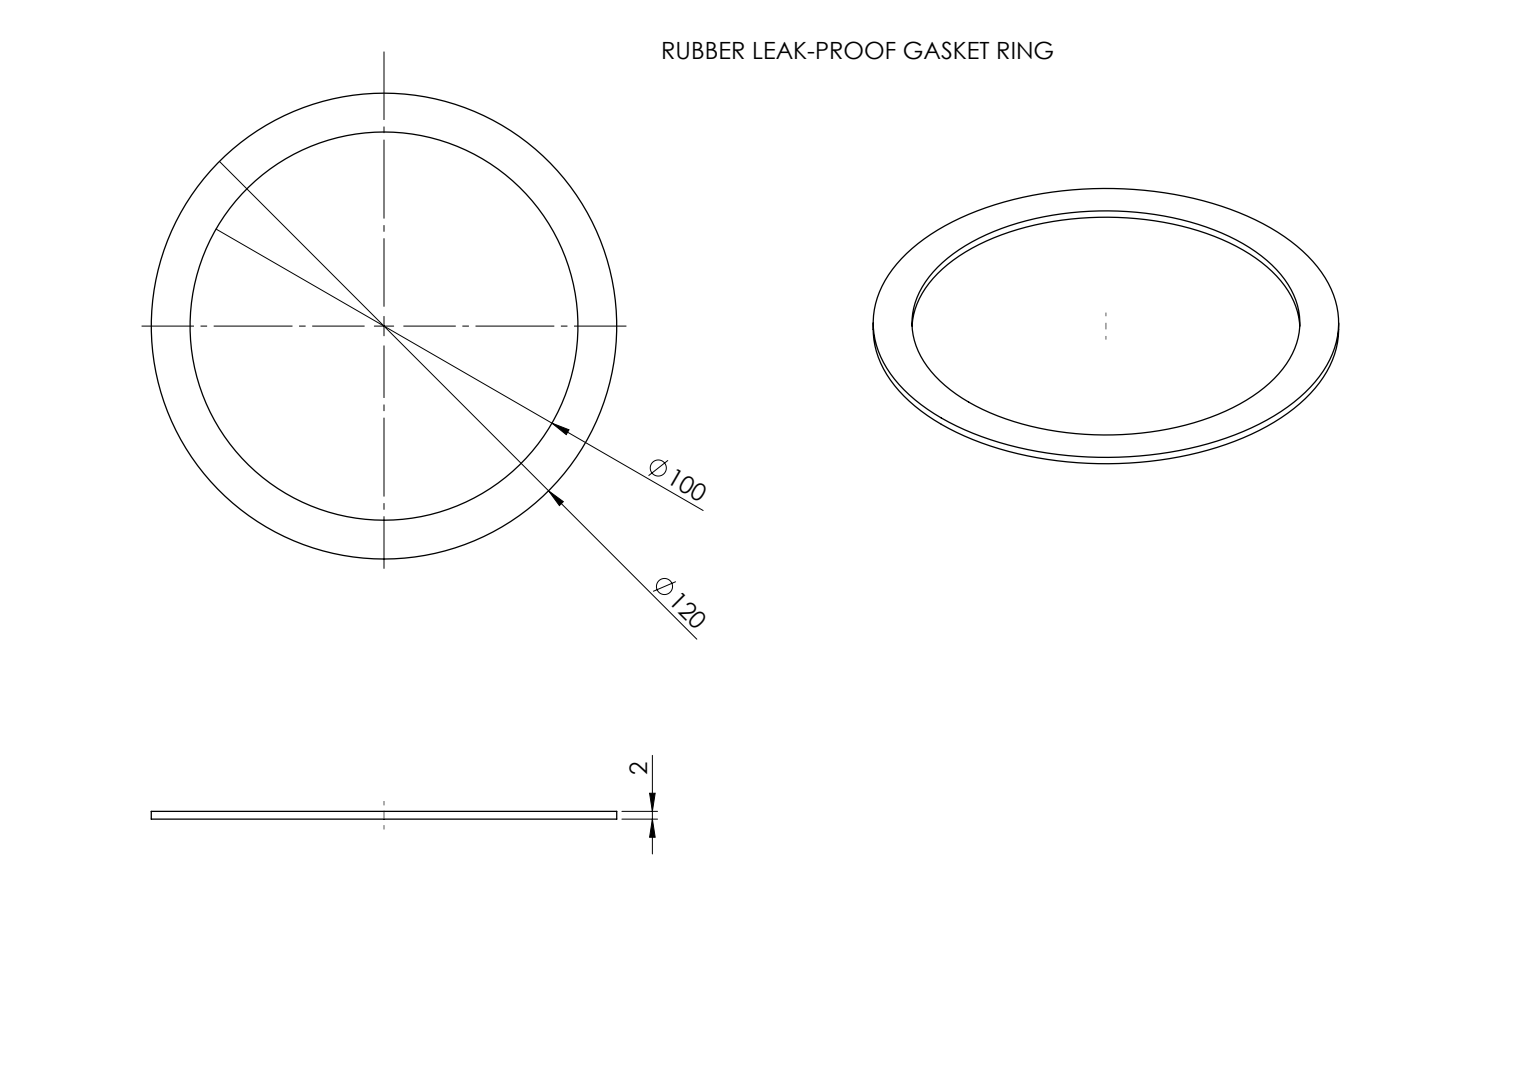
ISO-10303-21;
HEADER;
FILE_DESCRIPTION (('STEP AP214'),
    '1' );
FILE_NAME ('Rubber Leak-Proof Gasket Ring.step',
    '2026-10-09T15:02:13',
    ( '' ),
    ( '' ),
    'SwSTEP 2.0',
    'SolidWorks 2026',
    '' );
FILE_SCHEMA (( 'AUTOMOTIVE_DESIGN' ));
ENDSEC;

DATA;
#75=VERTEX_POINT ( 'NONE', #14029 ) ;
#118=ORIENTED_EDGE ( 'NONE', *, *, #603, .F. ) ;
#141=DIRECTION ( 'NONE',  ( 0.000000000000000000, 0.000000000000000000, -1.000000000000000000 ) ) ;
#205=EDGE_CURVE ( 'NONE', #75, #14665, #7073, .T. ) ;
#230=DIRECTION ( 'NONE',  ( 0.000000000000000000, 0.000000000000000000, 1.000000000000000000 ) ) ;
#240=DIRECTION ( 'NONE',  ( 0.000000000000000000, 1.000000000000000000, 0.000000000000000000 ) ) ;
#243=VERTEX_POINT ( 'NONE', #6253 ) ;
#295=PRODUCT_DEFINITION ( 'UNKNOWN', '', #14486, #8928 ) ;
#378=FACE_OUTER_BOUND ( 'NONE', #6121, .T. ) ;
#382=CARTESIAN_POINT ( 'NONE',  ( 0.000000000000000000, 52.00000000000000711, 0.000000000000000000 ) ) ;
#550=DIRECTION ( 'NONE',  ( 0.000000000000000000, 1.000000000000000000, 0.000000000000000000 ) ) ;
#603=EDGE_CURVE ( 'NONE', #14587, #8799, #10009, .T. ) ;
#730=SHAPE_REPRESENTATION_RELATIONSHIP ( 'NONE' , 'NONE' ,  #15829, #9194 ) ;
#848=DIRECTION ( 'NONE',  ( 0.000000000000000000, 0.000000000000000000, 1.000000000000000000 ) ) ;
#911=CYLINDRICAL_SURFACE ( 'NONE', #979, 50.00000000000000000 ) ;
#976=( LENGTH_UNIT ( ) NAMED_UNIT ( * ) SI_UNIT ( .MILLI., .METRE. ) );
#979=AXIS2_PLACEMENT_3D ( 'NONE', #3337, #9656, #12404 ) ;
#1079=ADVANCED_FACE ( 'NONE', ( #8408 ), #911, .F. ) ;
#1119=CIRCLE ( 'NONE', #15991, 50.00000000000000000 ) ;
#1131=AXIS2_PLACEMENT_3D ( 'NONE', #1874, #6969, #10701 ) ;
#1133=( NAMED_UNIT ( * ) PLANE_ANGLE_UNIT ( ) SI_UNIT ( $, .RADIAN. ) );
#1217=CIRCLE ( 'NONE', #4436, 50.00000000000000000 ) ;
#1229=EDGE_CURVE ( 'NONE', #8799, #14587, #16125, .T. ) ;
#1243=CIRCLE ( 'NONE', #5001, 50.00000000000000000 ) ;
#1279=CARTESIAN_POINT ( 'NONE',  ( 0.000000000000000000, 50.00000000000000000, 0.000000000000000000 ) ) ;
#1353=ORIENTED_EDGE ( 'NONE', *, *, #4912, .T. ) ;
#1385=CARTESIAN_POINT ( 'NONE',  ( 0.000000000000000000, 52.00000000000000711, -60.00000000000000711 ) ) ;
#1481=DIRECTION ( 'NONE',  ( -0.000000000000000000, -1.000000000000000000, -0.000000000000000000 ) ) ;
#1534=ADVANCED_FACE ( 'NONE', ( #5816, #3149 ), #10883, .T. ) ;
#1684=EDGE_CURVE ( 'NONE', #8698, #14922, #1243, .T. ) ;
#1738=( GEOMETRIC_REPRESENTATION_CONTEXT ( 3 ) GLOBAL_UNCERTAINTY_ASSIGNED_CONTEXT ( ( #14556 ) ) GLOBAL_UNIT_ASSIGNED_CONTEXT ( ( #9391, #6750, #13366 ) ) REPRESENTATION_CONTEXT ( 'NONE', 'WORKASPACE' ) );
#1874=CARTESIAN_POINT ( 'NONE',  ( 0.000000000000000000, 52.00000000000000711, 0.000000000000000000 ) ) ;
#1973=ORIENTED_EDGE ( 'NONE', *, *, #10109, .F. ) ;
#2000=EDGE_LOOP ( 'NONE', ( #3155, #11326, #2184, #1973 ) ) ;
#2077=APPLICATION_CONTEXT ( 'automotive_design' ) ;
#2158=CARTESIAN_POINT ( 'NONE',  ( 0.000000000000000000, 0.000000000000000000, 0.000000000000000000 ) ) ;
#2184=ORIENTED_EDGE ( 'NONE', *, *, #1684, .F. ) ;
#2306=AXIS2_PLACEMENT_3D ( 'NONE', #10308, #1481, #141 ) ;
#2469=VECTOR ( 'NONE', #6768, 1000.000000000000000 ) ;
#2506=LINE ( 'NONE', #11570, #11062 ) ;
#2528=PLANE ( 'NONE',  #6500 ) ;
#2581=AXIS2_PLACEMENT_3D ( 'NONE', #15699, #240, #10476 ) ;
#2725=CYLINDRICAL_SURFACE ( 'NONE', #2306, 60.00000000000000711 ) ;
#2829=DIRECTION ( 'NONE',  ( 0.000000000000000000, 1.000000000000000000, 0.000000000000000000 ) ) ;
#2954=ORIENTED_EDGE ( 'NONE', *, *, #14421, .T. ) ;
#3147=( NAMED_UNIT ( * ) PLANE_ANGLE_UNIT ( ) SI_UNIT ( $, .RADIAN. ) );
#3149=FACE_BOUND ( 'NONE', #5769, .T. ) ;
#3155=ORIENTED_EDGE ( 'NONE', *, *, #4858, .T. ) ;
#3337=CARTESIAN_POINT ( 'NONE',  ( 0.000000000000000000, 52.00000000000000711, 0.000000000000000000 ) ) ;
#3399=ADVANCED_FACE ( 'NONE', ( #10311 ), #8889, .F. ) ;
#3554=ORIENTED_EDGE ( 'NONE', *, *, #14421, .F. ) ;
#3656=SURFACE_STYLE_FILL_AREA ( #12620 ) ;
#3680=DIRECTION ( 'NONE',  ( 0.000000000000000000, 1.000000000000000000, 0.000000000000000000 ) ) ;
#3792=MECHANICAL_DESIGN_GEOMETRIC_PRESENTATION_REPRESENTATION('',(#10950),#14656);
#3875=STYLED_ITEM ( 'NONE', ( #9556 ), #9194 ) ;
#3944=ORIENTED_EDGE ( 'NONE', *, *, #12365, .F. ) ;
#4056=COLOUR_RGB ( '', 0.66274510, 0.83137255, 0.94901961) ;
#4226=SHAPE_DEFINITION_REPRESENTATION ( #11839, #15829 ) ;
#4230=DIRECTION ( 'NONE',  ( 0.000000000000000000, 0.000000000000000000, -1.000000000000000000 ) ) ;
#4436=AXIS2_PLACEMENT_3D ( 'NONE', #9671, #7184, #848 ) ;
#4466=LINE ( 'NONE', #9443, #4960 ) ;
#4525=ORIENTED_EDGE ( 'NONE', *, *, #205, .F. ) ;
#4541=ORIENTED_EDGE ( 'NONE', *, *, #14844, .T. ) ;
#4715=AXIS2_PLACEMENT_3D ( 'NONE', #13895, #6517, #10172 ) ;
#4752=( NAMED_UNIT ( * ) SI_UNIT ( $, .STERADIAN. ) SOLID_ANGLE_UNIT ( ) );
#4828=FILL_AREA_STYLE ('',( #13533 ) ) ;
#4858=EDGE_CURVE ( 'NONE', #243, #15421, #1217, .T. ) ;
#4912=EDGE_CURVE ( 'NONE', #14665, #14587, #2506, .T. ) ;
#4960=VECTOR ( 'NONE', #6023, 1000.000000000000000 ) ;
#5001=AXIS2_PLACEMENT_3D ( 'NONE', #5654, #2829, #13215 ) ;
#5190=CARTESIAN_POINT ( 'NONE',  ( 6.123233995736766085E-15, 52.00000000000000711, 50.00000000000000000 ) ) ;
#5227=CLOSED_SHELL ( 'NONE', ( #3399, #12072, #1534, #7840, #14756, #1079 ) ) ;
#5446=ORIENTED_EDGE ( 'NONE', *, *, #12365, .T. ) ;
#5480=CYLINDRICAL_SURFACE ( 'NONE', #14924, 60.00000000000000711 ) ;
#5621=PRODUCT ( 'Rubber Leak-Proof Gasket Ring', 'Rubber Leak-Proof Gasket Ring', '', ( #10375 ) ) ;
#5654=CARTESIAN_POINT ( 'NONE',  ( 0.000000000000000000, 50.00000000000000000, 0.000000000000000000 ) ) ;
#5769=EDGE_LOOP ( 'NONE', ( #6079, #3944 ) ) ;
#5816=FACE_OUTER_BOUND ( 'NONE', #9542, .T. ) ;
#5897=( NAMED_UNIT ( * ) SI_UNIT ( $, .STERADIAN. ) SOLID_ANGLE_UNIT ( ) );
#5982=DIRECTION ( 'NONE',  ( 0.000000000000000000, 1.000000000000000000, 0.000000000000000000 ) ) ;
#6023=DIRECTION ( 'NONE',  ( -0.000000000000000000, -1.000000000000000000, -0.000000000000000000 ) ) ;
#6071=SURFACE_SIDE_STYLE ('',( #14856 ) ) ;
#6079=ORIENTED_EDGE ( 'NONE', *, *, #4858, .F. ) ;
#6121=EDGE_LOOP ( 'NONE', ( #7382, #6800, #1353, #10798 ) ) ;
#6149=SURFACE_STYLE_USAGE ( .BOTH. , #12538 ) ;
#6253=CARTESIAN_POINT ( 'NONE',  ( 0.000000000000000000, 52.00000000000000711, -50.00000000000000000 ) ) ;
#6369=DIRECTION ( 'NONE',  ( 0.000000000000000000, 1.000000000000000000, 0.000000000000000000 ) ) ;
#6500=AXIS2_PLACEMENT_3D ( 'NONE', #1279, #6369, #10186 ) ;
#6517=DIRECTION ( 'NONE',  ( 0.000000000000000000, 1.000000000000000000, 0.000000000000000000 ) ) ;
#6573=EDGE_LOOP ( 'NONE', ( #118, #13201 ) ) ;
#6615=UNCERTAINTY_MEASURE_WITH_UNIT (LENGTH_MEASURE( 1.000000000000000082E-05 ), #12209, 'distance_accuracy_value', 'NONE');
#6750=( NAMED_UNIT ( * ) PLANE_ANGLE_UNIT ( ) SI_UNIT ( $, .RADIAN. ) );
#6768=DIRECTION ( 'NONE',  ( -0.000000000000000000, -1.000000000000000000, -0.000000000000000000 ) ) ;
#6800=ORIENTED_EDGE ( 'NONE', *, *, #14844, .F. ) ;
#6969=DIRECTION ( 'NONE',  ( 0.000000000000000000, 1.000000000000000000, 0.000000000000000000 ) ) ;
#6984=CARTESIAN_POINT ( 'NONE',  ( 0.000000000000000000, 50.00000000000000000, 0.000000000000000000 ) ) ;
#7073=CIRCLE ( 'NONE', #11325, 60.00000000000000711 ) ;
#7100=UNCERTAINTY_MEASURE_WITH_UNIT (LENGTH_MEASURE( 1.000000000000000082E-05 ), #976, 'distance_accuracy_value', 'NONE');
#7184=DIRECTION ( 'NONE',  ( 0.000000000000000000, 1.000000000000000000, 0.000000000000000000 ) ) ;
#7228=FILL_AREA_STYLE_COLOUR ( '', #4056 ) ;
#7382=ORIENTED_EDGE ( 'NONE', *, *, #15572, .F. ) ;
#7475=ORIENTED_EDGE ( 'NONE', *, *, #1229, .T. ) ;
#7631=AXIS2_PLACEMENT_3D ( 'NONE', #7886, #550, #230 ) ;
#7828=LINE ( 'NONE', #12903, #2469 ) ;
#7840=ADVANCED_FACE ( 'NONE', ( #8849, #13909 ), #2528, .F. ) ;
#7865=EDGE_LOOP ( 'NONE', ( #4525, #11866, #7475, #14355 ) ) ;
#7886=CARTESIAN_POINT ( 'NONE',  ( 0.000000000000000000, 52.00000000000000711, 0.000000000000000000 ) ) ;
#7957=AXIS2_PLACEMENT_3D ( 'NONE', #12549, #12717, #15367 ) ;
#8006=DIRECTION ( 'NONE',  ( -0.000000000000000000, -1.000000000000000000, -0.000000000000000000 ) ) ;
#8178=LINE ( 'NONE', #10600, #15299 ) ;
#8221=SURFACE_STYLE_USAGE ( .BOTH. , #6071 ) ;
#8223=CARTESIAN_POINT ( 'NONE',  ( 0.000000000000000000, 52.00000000000000711, 0.000000000000000000 ) ) ;
#8312=CIRCLE ( 'NONE', #1131, 60.00000000000000711 ) ;
#8408=FACE_OUTER_BOUND ( 'NONE', #10218, .T. ) ;
#8560=DIRECTION ( 'NONE',  ( 1.000000000000000000, 0.000000000000000000, 0.000000000000000000 ) ) ;
#8698=VERTEX_POINT ( 'NONE', #10157 ) ;
#8799=VERTEX_POINT ( 'NONE', #9247 ) ;
#8849=FACE_OUTER_BOUND ( 'NONE', #6573, .T. ) ;
#8889=CYLINDRICAL_SURFACE ( 'NONE', #7957, 50.00000000000000000 ) ;
#8928=PRODUCT_DEFINITION_CONTEXT ( 'detailed design', #2077, 'design' ) ;
#9178=( GEOMETRIC_REPRESENTATION_CONTEXT ( 3 ) GLOBAL_UNCERTAINTY_ASSIGNED_CONTEXT ( ( #6615 ) ) GLOBAL_UNIT_ASSIGNED_CONTEXT ( ( #12209, #3147, #5897 ) ) REPRESENTATION_CONTEXT ( 'NONE', 'WORKASPACE' ) );
#9194=ADVANCED_BREP_SHAPE_REPRESENTATION ( '', ( #14597, #15812 ), #1738 ) ;
#9247=CARTESIAN_POINT ( 'NONE',  ( 7.347880794884119933E-15, 50.00000000000000000, 60.00000000000000711 ) ) ;
#9391=( LENGTH_UNIT ( ) NAMED_UNIT ( * ) SI_UNIT ( .MILLI., .METRE. ) );
#9443=CARTESIAN_POINT ( 'NONE',  ( 0.000000000000000000, 52.00000000000000711, -50.00000000000000000 ) ) ;
#9487=EDGE_LOOP ( 'NONE', ( #10083, #2954 ) ) ;
#9542=EDGE_LOOP ( 'NONE', ( #4541, #12694 ) ) ;
#9556=PRESENTATION_STYLE_ASSIGNMENT (( #8221 ) ) ;
#9656=DIRECTION ( 'NONE',  ( -0.000000000000000000, -1.000000000000000000, -0.000000000000000000 ) ) ;
#9671=CARTESIAN_POINT ( 'NONE',  ( 0.000000000000000000, 52.00000000000000711, 0.000000000000000000 ) ) ;
#9700=CARTESIAN_POINT ( 'NONE',  ( 6.123233995736766085E-15, 50.00000000000000000, 50.00000000000000000 ) ) ;
#9720=CIRCLE ( 'NONE', #7631, 50.00000000000000000 ) ;
#10009=CIRCLE ( 'NONE', #4715, 60.00000000000000711 ) ;
#10083=ORIENTED_EDGE ( 'NONE', *, *, #1684, .T. ) ;
#10109=EDGE_CURVE ( 'NONE', #243, #8698, #4466, .T. ) ;
#10157=CARTESIAN_POINT ( 'NONE',  ( 0.000000000000000000, 50.00000000000000000, -50.00000000000000000 ) ) ;
#10172=DIRECTION ( 'NONE',  ( 0.000000000000000000, 0.000000000000000000, 1.000000000000000000 ) ) ;
#10186=DIRECTION ( 'NONE',  ( 0.000000000000000000, -0.000000000000000000, 1.000000000000000000 ) ) ;
#10218=EDGE_LOOP ( 'NONE', ( #15788, #5446, #15922, #3554 ) ) ;
#10308=CARTESIAN_POINT ( 'NONE',  ( 0.000000000000000000, 52.00000000000000711, 0.000000000000000000 ) ) ;
#10311=FACE_OUTER_BOUND ( 'NONE', #2000, .T. ) ;
#10375=PRODUCT_CONTEXT ( 'NONE', #12159, 'mechanical' ) ;
#10476=DIRECTION ( 'NONE',  ( 0.000000000000000000, 0.000000000000000000, 1.000000000000000000 ) ) ;
#10552=CARTESIAN_POINT ( 'NONE',  ( 0.000000000000000000, 52.00000000000000711, 0.000000000000000000 ) ) ;
#10600=CARTESIAN_POINT ( 'NONE',  ( 6.123233995736766085E-15, 52.00000000000000711, 50.00000000000000000 ) ) ;
#10701=DIRECTION ( 'NONE',  ( 0.000000000000000000, 0.000000000000000000, 1.000000000000000000 ) ) ;
#10798=ORIENTED_EDGE ( 'NONE', *, *, #603, .T. ) ;
#10811=DIRECTION ( 'NONE',  ( 0.000000000000000000, 1.000000000000000000, 0.000000000000000000 ) ) ;
#10883=PLANE ( 'NONE',  #12938 ) ;
#10950=STYLED_ITEM ( 'NONE', ( #16122 ), #14597 ) ;
#11037=COLOUR_RGB ( '', 0.66274510, 0.83137255, 0.94901961) ;
#11062=VECTOR ( 'NONE', #15308, 1000.000000000000000 ) ;
#11073=DIRECTION ( 'NONE',  ( 0.000000000000000000, 0.000000000000000000, 1.000000000000000000 ) ) ;
#11104=EDGE_CURVE ( 'NONE', #15421, #14922, #8178, .T. ) ;
#11325=AXIS2_PLACEMENT_3D ( 'NONE', #382, #3680, #13721 ) ;
#11326=ORIENTED_EDGE ( 'NONE', *, *, #11104, .T. ) ;
#11390=FACE_OUTER_BOUND ( 'NONE', #7865, .T. ) ;
#11570=CARTESIAN_POINT ( 'NONE',  ( 0.000000000000000000, 52.00000000000000711, -60.00000000000000711 ) ) ;
#11839=PRODUCT_DEFINITION_SHAPE ( 'NONE', 'NONE',  #295 ) ;
#11866=ORIENTED_EDGE ( 'NONE', *, *, #15572, .T. ) ;
#12072=ADVANCED_FACE ( 'NONE', ( #11390 ), #2725, .T. ) ;
#12159=APPLICATION_CONTEXT ( 'automotive_design' ) ;
#12209=( LENGTH_UNIT ( ) NAMED_UNIT ( * ) SI_UNIT ( .MILLI., .METRE. ) );
#12365=EDGE_CURVE ( 'NONE', #15421, #243, #9720, .T. ) ;
#12404=DIRECTION ( 'NONE',  ( 0.000000000000000000, 0.000000000000000000, -1.000000000000000000 ) ) ;
#12464=CARTESIAN_POINT ( 'NONE',  ( 0.000000000000000000, 50.00000000000000000, -60.00000000000000711 ) ) ;
#12538=SURFACE_SIDE_STYLE ('',( #3656 ) ) ;
#12549=CARTESIAN_POINT ( 'NONE',  ( 0.000000000000000000, 52.00000000000000711, 0.000000000000000000 ) ) ;
#12620=FILL_AREA_STYLE ('',( #7228 ) ) ;
#12694=ORIENTED_EDGE ( 'NONE', *, *, #205, .T. ) ;
#12717=DIRECTION ( 'NONE',  ( -0.000000000000000000, -1.000000000000000000, -0.000000000000000000 ) ) ;
#12903=CARTESIAN_POINT ( 'NONE',  ( 7.347880794884119933E-15, 52.00000000000000711, 60.00000000000000711 ) ) ;
#12938=AXIS2_PLACEMENT_3D ( 'NONE', #8223, #5982, #13289 ) ;
#13159=MECHANICAL_DESIGN_GEOMETRIC_PRESENTATION_REPRESENTATION('',(#3875),#9178);
#13201=ORIENTED_EDGE ( 'NONE', *, *, #1229, .F. ) ;
#13215=DIRECTION ( 'NONE',  ( 0.000000000000000000, 0.000000000000000000, 1.000000000000000000 ) ) ;
#13289=DIRECTION ( 'NONE',  ( 0.000000000000000000, -0.000000000000000000, 1.000000000000000000 ) ) ;
#13366=( NAMED_UNIT ( * ) SI_UNIT ( $, .STERADIAN. ) SOLID_ANGLE_UNIT ( ) );
#13533=FILL_AREA_STYLE_COLOUR ( '', #11037 ) ;
#13721=DIRECTION ( 'NONE',  ( 0.000000000000000000, 0.000000000000000000, 1.000000000000000000 ) ) ;
#13895=CARTESIAN_POINT ( 'NONE',  ( 0.000000000000000000, 50.00000000000000000, 0.000000000000000000 ) ) ;
#13909=FACE_BOUND ( 'NONE', #9487, .T. ) ;
#14029=CARTESIAN_POINT ( 'NONE',  ( 7.347880794884119933E-15, 52.00000000000000711, 60.00000000000000711 ) ) ;
#14355=ORIENTED_EDGE ( 'NONE', *, *, #4912, .F. ) ;
#14421=EDGE_CURVE ( 'NONE', #14922, #8698, #1119, .T. ) ;
#14486=PRODUCT_DEFINITION_FORMATION_WITH_SPECIFIED_SOURCE ( 'ANY', '', #5621, .NOT_KNOWN. ) ;
#14556=UNCERTAINTY_MEASURE_WITH_UNIT (LENGTH_MEASURE( 1.000000000000000082E-05 ), #9391, 'distance_accuracy_value', 'NONE');
#14587=VERTEX_POINT ( 'NONE', #12464 ) ;
#14597=MANIFOLD_SOLID_BREP ( 'Boss-Extrude1', #5227 ) ;
#14656=( GEOMETRIC_REPRESENTATION_CONTEXT ( 3 ) GLOBAL_UNCERTAINTY_ASSIGNED_CONTEXT ( ( #7100 ) ) GLOBAL_UNIT_ASSIGNED_CONTEXT ( ( #976, #1133, #4752 ) ) REPRESENTATION_CONTEXT ( 'NONE', 'WORKASPACE' ) );
#14665=VERTEX_POINT ( 'NONE', #1385 ) ;
#14756=ADVANCED_FACE ( 'NONE', ( #378 ), #5480, .T. ) ;
#14844=EDGE_CURVE ( 'NONE', #14665, #75, #8312, .T. ) ;
#14856=SURFACE_STYLE_FILL_AREA ( #4828 ) ;
#14922=VERTEX_POINT ( 'NONE', #9700 ) ;
#14924=AXIS2_PLACEMENT_3D ( 'NONE', #10552, #15608, #4230 ) ;
#15299=VECTOR ( 'NONE', #8006, 1000.000000000000000 ) ;
#15308=DIRECTION ( 'NONE',  ( -0.000000000000000000, -1.000000000000000000, -0.000000000000000000 ) ) ;
#15367=DIRECTION ( 'NONE',  ( 0.000000000000000000, 0.000000000000000000, -1.000000000000000000 ) ) ;
#15421=VERTEX_POINT ( 'NONE', #5190 ) ;
#15572=EDGE_CURVE ( 'NONE', #75, #8799, #7828, .T. ) ;
#15608=DIRECTION ( 'NONE',  ( -0.000000000000000000, -1.000000000000000000, -0.000000000000000000 ) ) ;
#15699=CARTESIAN_POINT ( 'NONE',  ( 0.000000000000000000, 50.00000000000000000, 0.000000000000000000 ) ) ;
#15788=ORIENTED_EDGE ( 'NONE', *, *, #11104, .F. ) ;
#15812=AXIS2_PLACEMENT_3D ( 'NONE', #2158, #11073, #8560 ) ;
#15829=SHAPE_REPRESENTATION ( 'Rubber Leak-Proof Gasket Ring', ( #15812 ), #1738 ) ;
#15874=DIRECTION ( 'NONE',  ( 0.000000000000000000, 0.000000000000000000, 1.000000000000000000 ) ) ;
#15922=ORIENTED_EDGE ( 'NONE', *, *, #10109, .T. ) ;
#15991=AXIS2_PLACEMENT_3D ( 'NONE', #6984, #10811, #15874 ) ;
#16122=PRESENTATION_STYLE_ASSIGNMENT (( #6149 ) ) ;
#16125=CIRCLE ( 'NONE', #2581, 60.00000000000000711 ) ;
ENDSEC;
END-ISO-10303-21;
